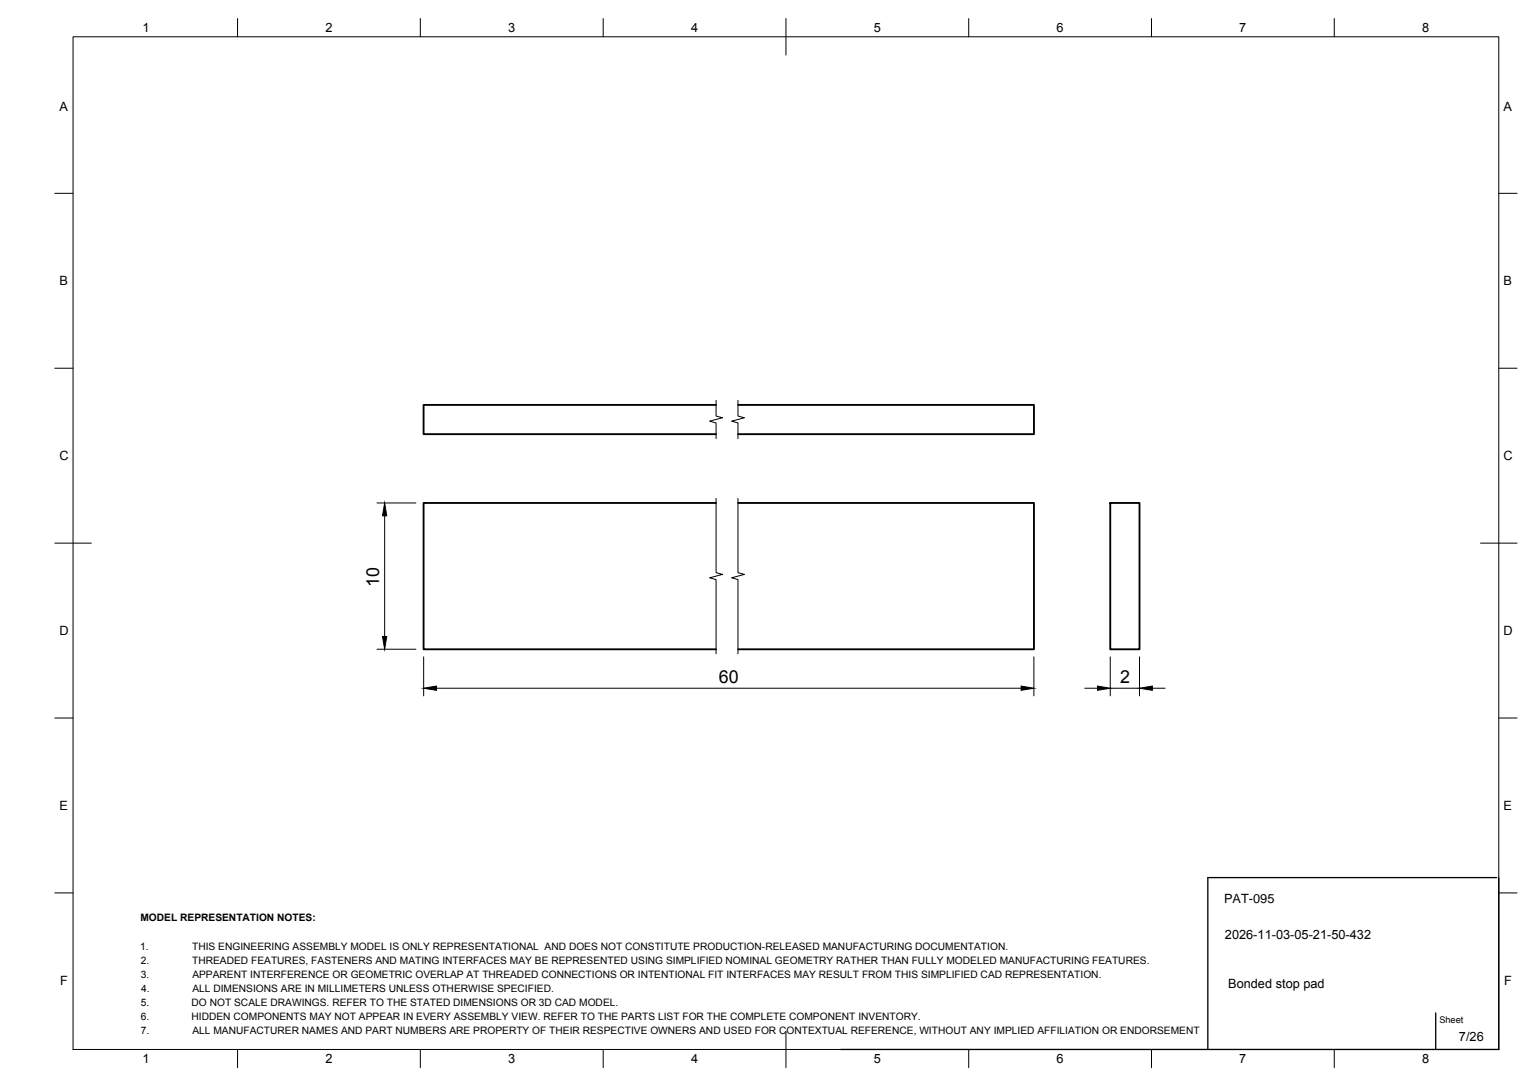
ISO-10303-21;
HEADER;
/* Generated by software containing ST-Developer
 * from STEP Tools, Inc. (www.steptools.com) 
 */

FILE_DESCRIPTION(
/* description */ ('Single-Axis Profile-Rail Linear Slide'),
/* implementation_level */ '2;1');

FILE_NAME(
/* name */ 'Bonded stop pad.step',
/* time_stamp */ '2026-10-27T10:47:43-07:00',
/* author */ (''),
/* organization */ (''),
/* preprocessor_version */ 'ST-DEVELOPER v20.2',
/* originating_system */ 'Autodesk Translation Framework v15.17.0.0',
/* authorisation */ '');

FILE_SCHEMA (('AUTOMOTIVE_DESIGN { 1 0 10303 214 3 1 1 }'));
ENDSEC;

DATA;
#10=MECHANICAL_DESIGN_GEOMETRIC_PRESENTATION_REPRESENTATION('',(#331),#14478);
#277=SHAPE_REPRESENTATION_RELATIONSHIP('SRR','None',#14607,#304);
#304=ADVANCED_BREP_SHAPE_REPRESENTATION('',(#358),#14451);
#331=STYLED_ITEM('',(#14845),#358);
#358=MANIFOLD_SOLID_BREP('Body1',#8591);
#482=PLANE('',#8992);
#483=PLANE('',#8993);
#484=PLANE('',#8994);
#485=PLANE('',#8995);
#486=PLANE('',#8996);
#487=PLANE('',#8997);
#872=FACE_OUTER_BOUND('',#1361,.T.);
#873=FACE_OUTER_BOUND('',#1362,.T.);
#874=FACE_OUTER_BOUND('',#1363,.T.);
#875=FACE_OUTER_BOUND('',#1364,.T.);
#876=FACE_OUTER_BOUND('',#1365,.T.);
#877=FACE_OUTER_BOUND('',#1366,.T.);
#1361=EDGE_LOOP('',(#5969,#5970,#5971,#5972));
#1362=EDGE_LOOP('',(#5973,#5974,#5975,#5976));
#1363=EDGE_LOOP('',(#5977,#5978,#5979,#5980));
#1364=EDGE_LOOP('',(#5981,#5982,#5983,#5984));
#1365=EDGE_LOOP('',(#5985,#5986,#5987,#5988));
#1366=EDGE_LOOP('',(#5989,#5990,#5991,#5992));
#1882=LINE('',#12166,#2853);
#1883=LINE('',#12168,#2854);
#1884=LINE('',#12170,#2855);
#1885=LINE('',#12171,#2856);
#1886=LINE('',#12174,#2857);
#1887=LINE('',#12176,#2858);
#1888=LINE('',#12177,#2859);
#1889=LINE('',#12180,#2860);
#1890=LINE('',#12182,#2861);
#1891=LINE('',#12183,#2862);
#1892=LINE('',#12185,#2863);
#1893=LINE('',#12186,#2864);
#2853=VECTOR('',#9811,1.);
#2854=VECTOR('',#9812,1.);
#2855=VECTOR('',#9813,1.);
#2856=VECTOR('',#9814,1.);
#2857=VECTOR('',#9817,1.);
#2858=VECTOR('',#9818,1.);
#2859=VECTOR('',#9819,1.);
#2860=VECTOR('',#9822,1.);
#2861=VECTOR('',#9823,1.);
#2862=VECTOR('',#9824,1.);
#2863=VECTOR('',#9827,1.);
#2864=VECTOR('',#9828,1.);
#3990=VERTEX_POINT('',#12164);
#3991=VERTEX_POINT('',#12165);
#3992=VERTEX_POINT('',#12167);
#3993=VERTEX_POINT('',#12169);
#3994=VERTEX_POINT('',#12173);
#3995=VERTEX_POINT('',#12175);
#3996=VERTEX_POINT('',#12179);
#3997=VERTEX_POINT('',#12181);
#4762=EDGE_CURVE('',#3990,#3991,#1882,.T.);
#4763=EDGE_CURVE('',#3991,#3992,#1883,.T.);
#4764=EDGE_CURVE('',#3993,#3992,#1884,.T.);
#4765=EDGE_CURVE('',#3990,#3993,#1885,.T.);
#4766=EDGE_CURVE('',#3994,#3990,#1886,.T.);
#4767=EDGE_CURVE('',#3995,#3993,#1887,.T.);
#4768=EDGE_CURVE('',#3994,#3995,#1888,.T.);
#4769=EDGE_CURVE('',#3996,#3994,#1889,.T.);
#4770=EDGE_CURVE('',#3997,#3995,#1890,.T.);
#4771=EDGE_CURVE('',#3996,#3997,#1891,.T.);
#4772=EDGE_CURVE('',#3991,#3996,#1892,.T.);
#4773=EDGE_CURVE('',#3992,#3997,#1893,.T.);
#5969=ORIENTED_EDGE('',*,*,#4762,.T.);
#5970=ORIENTED_EDGE('',*,*,#4763,.T.);
#5971=ORIENTED_EDGE('',*,*,#4764,.F.);
#5972=ORIENTED_EDGE('',*,*,#4765,.F.);
#5973=ORIENTED_EDGE('',*,*,#4766,.T.);
#5974=ORIENTED_EDGE('',*,*,#4765,.T.);
#5975=ORIENTED_EDGE('',*,*,#4767,.F.);
#5976=ORIENTED_EDGE('',*,*,#4768,.F.);
#5977=ORIENTED_EDGE('',*,*,#4769,.T.);
#5978=ORIENTED_EDGE('',*,*,#4768,.T.);
#5979=ORIENTED_EDGE('',*,*,#4770,.F.);
#5980=ORIENTED_EDGE('',*,*,#4771,.F.);
#5981=ORIENTED_EDGE('',*,*,#4772,.T.);
#5982=ORIENTED_EDGE('',*,*,#4771,.T.);
#5983=ORIENTED_EDGE('',*,*,#4773,.F.);
#5984=ORIENTED_EDGE('',*,*,#4763,.F.);
#5985=ORIENTED_EDGE('',*,*,#4773,.T.);
#5986=ORIENTED_EDGE('',*,*,#4770,.T.);
#5987=ORIENTED_EDGE('',*,*,#4767,.T.);
#5988=ORIENTED_EDGE('',*,*,#4764,.T.);
#5989=ORIENTED_EDGE('',*,*,#4772,.F.);
#5990=ORIENTED_EDGE('',*,*,#4762,.F.);
#5991=ORIENTED_EDGE('',*,*,#4766,.F.);
#5992=ORIENTED_EDGE('',*,*,#4769,.F.);
#8166=ADVANCED_FACE('',(#872),#482,.T.);
#8167=ADVANCED_FACE('',(#873),#483,.T.);
#8168=ADVANCED_FACE('',(#874),#484,.T.);
#8169=ADVANCED_FACE('',(#875),#485,.T.);
#8170=ADVANCED_FACE('',(#876),#486,.T.);
#8171=ADVANCED_FACE('',(#877),#487,.F.);
#8591=CLOSED_SHELL('',(#8166,#8167,#8168,#8169,#8170,#8171));
#8991=AXIS2_PLACEMENT_3D('',#12162,#9807,#9808);
#8992=AXIS2_PLACEMENT_3D('',#12163,#9809,#9810);
#8993=AXIS2_PLACEMENT_3D('',#12172,#9815,#9816);
#8994=AXIS2_PLACEMENT_3D('',#12178,#9820,#9821);
#8995=AXIS2_PLACEMENT_3D('',#12184,#9825,#9826);
#8996=AXIS2_PLACEMENT_3D('',#12187,#9829,#9830);
#8997=AXIS2_PLACEMENT_3D('',#12188,#9831,#9832);
#9807=DIRECTION('axis',(0.,0.,1.));
#9808=DIRECTION('refdir',(1.,0.,0.));
#9809=DIRECTION('center_axis',(0.,1.,0.));
#9810=DIRECTION('ref_axis',(-1.,0.,0.));
#9811=DIRECTION('',(-1.,0.,0.));
#9812=DIRECTION('',(0.,0.,1.));
#9813=DIRECTION('',(-1.,0.,0.));
#9814=DIRECTION('',(0.,0.,1.));
#9815=DIRECTION('center_axis',(1.,0.,0.));
#9816=DIRECTION('ref_axis',(0.,1.,0.));
#9817=DIRECTION('',(0.,1.,0.));
#9818=DIRECTION('',(0.,1.,0.));
#9819=DIRECTION('',(0.,0.,1.));
#9820=DIRECTION('center_axis',(0.,-1.,0.));
#9821=DIRECTION('ref_axis',(1.,0.,0.));
#9822=DIRECTION('',(1.,0.,0.));
#9823=DIRECTION('',(1.,0.,0.));
#9824=DIRECTION('',(0.,0.,1.));
#9825=DIRECTION('center_axis',(-1.,0.,0.));
#9826=DIRECTION('ref_axis',(0.,-1.,0.));
#9827=DIRECTION('',(0.,-1.,0.));
#9828=DIRECTION('',(0.,-1.,0.));
#9829=DIRECTION('center_axis',(0.,0.,1.));
#9830=DIRECTION('ref_axis',(1.,0.,0.));
#9831=DIRECTION('center_axis',(0.,0.,1.));
#9832=DIRECTION('ref_axis',(1.,0.,0.));
#12162=CARTESIAN_POINT('',(0.,0.,0.));
#12163=CARTESIAN_POINT('Origin',(0.2,3.,5.2));
#12164=CARTESIAN_POINT('',(0.2,3.,5.2));
#12165=CARTESIAN_POINT('',(0.,3.,5.2));
#12166=CARTESIAN_POINT('',(0.2,3.,5.2));
#12167=CARTESIAN_POINT('',(0.,3.,6.2));
#12168=CARTESIAN_POINT('',(0.,3.,5.2));
#12169=CARTESIAN_POINT('',(0.2,3.,6.2));
#12170=CARTESIAN_POINT('',(0.2,3.,6.2));
#12171=CARTESIAN_POINT('',(0.2,3.,5.2));
#12172=CARTESIAN_POINT('Origin',(0.2,-3.,5.2));
#12173=CARTESIAN_POINT('',(0.2,-3.,5.2));
#12174=CARTESIAN_POINT('',(0.2,-3.,5.2));
#12175=CARTESIAN_POINT('',(0.2,-3.,6.2));
#12176=CARTESIAN_POINT('',(0.2,-3.,6.2));
#12177=CARTESIAN_POINT('',(0.2,-3.,5.2));
#12178=CARTESIAN_POINT('Origin',(0.,-3.,5.2));
#12179=CARTESIAN_POINT('',(0.,-3.,5.2));
#12180=CARTESIAN_POINT('',(0.,-3.,5.2));
#12181=CARTESIAN_POINT('',(0.,-3.,6.2));
#12182=CARTESIAN_POINT('',(0.,-3.,6.2));
#12183=CARTESIAN_POINT('',(0.,-3.,5.2));
#12184=CARTESIAN_POINT('Origin',(0.,3.,5.2));
#12185=CARTESIAN_POINT('',(0.,3.,5.2));
#12186=CARTESIAN_POINT('',(0.,3.,6.2));
#12187=CARTESIAN_POINT('Origin',(0.1,0.,6.2));
#12188=CARTESIAN_POINT('Origin',(0.1,0.,5.2));
#14419=UNCERTAINTY_MEASURE_WITH_UNIT(LENGTH_MEASURE(0.001),#14479,
'DISTANCE_ACCURACY_VALUE',
'Maximum model space distance between geometric entities at asserted c
onnectivities');
#14446=UNCERTAINTY_MEASURE_WITH_UNIT(LENGTH_MEASURE(0.001),#14479,
'DISTANCE_ACCURACY_VALUE',
'Maximum model space distance between geometric entities at asserted c
onnectivities');
#14451=(
GEOMETRIC_REPRESENTATION_CONTEXT(3)
GLOBAL_UNCERTAINTY_ASSIGNED_CONTEXT((#14419))
GLOBAL_UNIT_ASSIGNED_CONTEXT((#14479,#14481,#14482))
REPRESENTATION_CONTEXT('','3D')
);
#14478=(
GEOMETRIC_REPRESENTATION_CONTEXT(3)
GLOBAL_UNCERTAINTY_ASSIGNED_CONTEXT((#14446))
GLOBAL_UNIT_ASSIGNED_CONTEXT((#14479,#14481,#14482))
REPRESENTATION_CONTEXT('','3D')
);
#14479=(
LENGTH_UNIT()
NAMED_UNIT(*)
SI_UNIT(.CENTI.,.METRE.)
);
#14481=(
NAMED_UNIT(*)
PLANE_ANGLE_UNIT()
SI_UNIT($,.RADIAN.)
);
#14482=(
NAMED_UNIT(*)
SI_UNIT($,.STERADIAN.)
SOLID_ANGLE_UNIT()
);
#14487=SHAPE_DEFINITION_REPRESENTATION(#14518,#14607);
#14518=PRODUCT_DEFINITION_SHAPE('',$,#14639);
#14607=SHAPE_REPRESENTATION('',(#8991),#14451);
#14634=PRODUCT_DEFINITION_CONTEXT('part definition',#14729,'design');
#14639=PRODUCT_DEFINITION('Bonded stop pad','Bonded stop pad',#14670,#14634);
#14670=PRODUCT_DEFINITION_FORMATION('',$,#14735);
#14729=APPLICATION_CONTEXT(
'Core Data for Automotive Mechanical Design Process');
#14730=PRODUCT_CONTEXT('part definition',#14729,'mechanical');
#14735=PRODUCT('Bonded stop pad','Bonded stop pad','Bonded stop pad',(#14730));
#14839=COLOUR_RGB('Off White',0.89,0.88,0.83);
#14840=FILL_AREA_STYLE_COLOUR('',#14839);
#14841=FILL_AREA_STYLE('',(#14840));
#14842=SURFACE_STYLE_FILL_AREA(#14841);
#14843=SURFACE_SIDE_STYLE('',(#14842));
#14844=SURFACE_STYLE_USAGE(.BOTH.,#14843);
#14845=PRESENTATION_STYLE_ASSIGNMENT((#14844));
ENDSEC;
END-ISO-10303-21;
